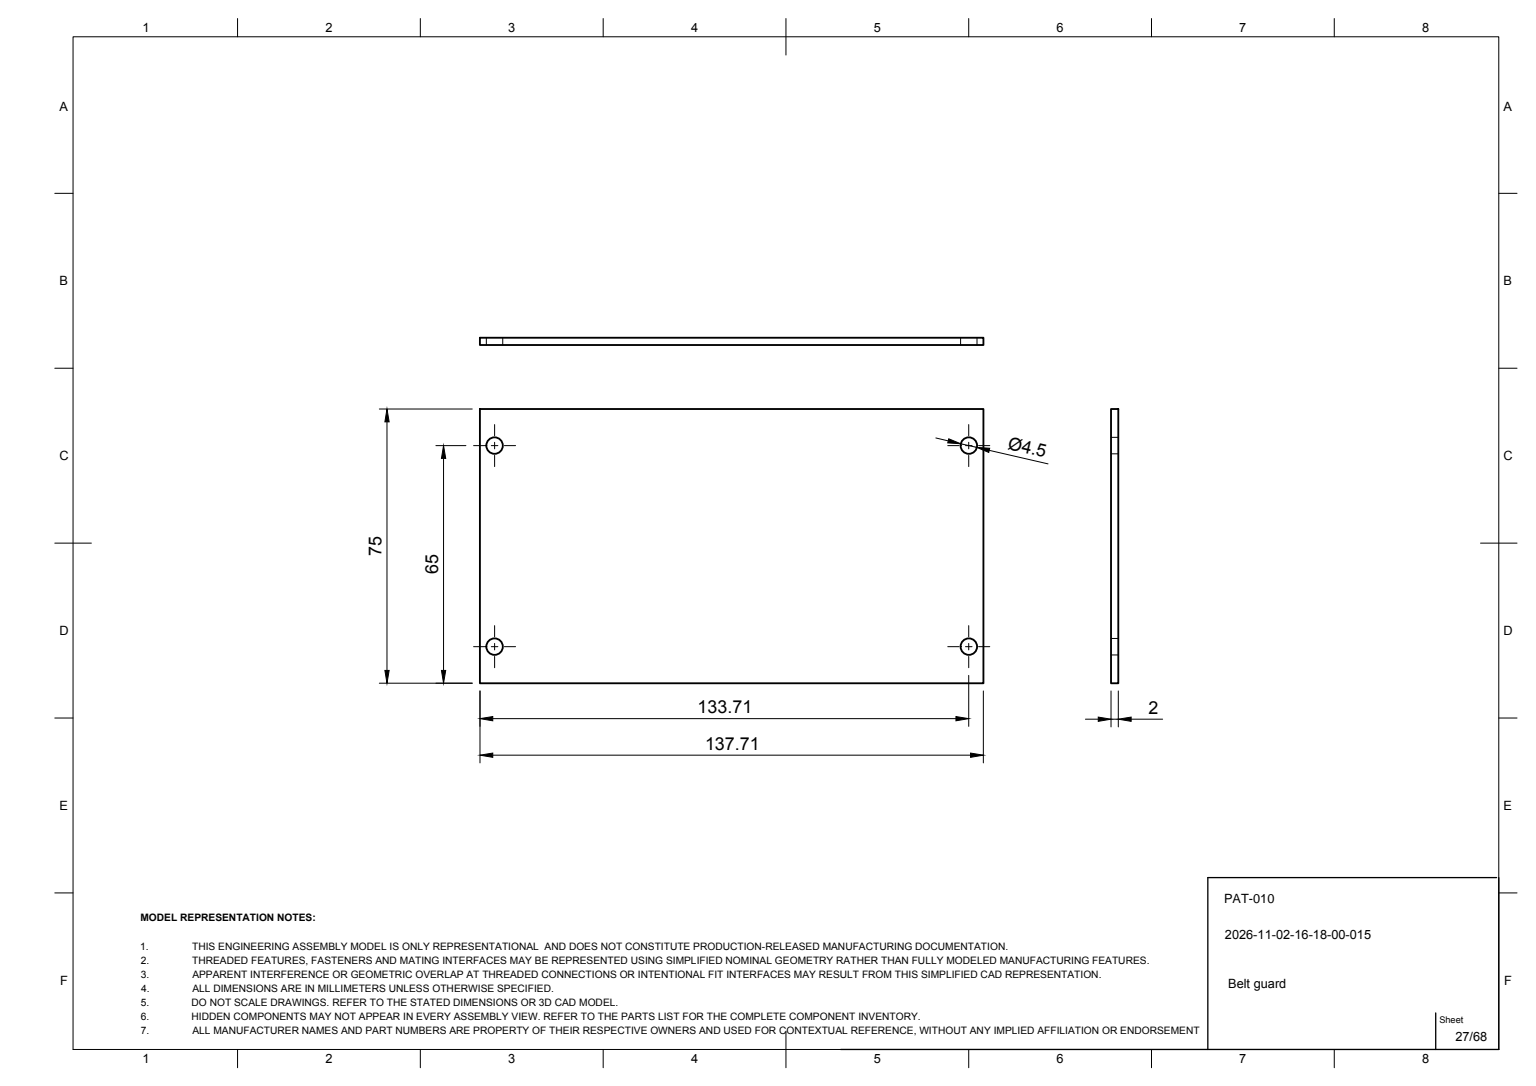
ISO-10303-21;
HEADER;
/* Generated by software containing ST-Developer
 * from STEP Tools, Inc. (www.steptools.com) 
 */

FILE_DESCRIPTION(
/* description */ ('Belt conveyor head drive unit'),
/* implementation_level */ '2;1');

FILE_NAME(
/* name */ 'Belt guard.step',
/* time_stamp */ '2026-10-28T03:26:19-07:00',
/* author */ (''),
/* organization */ (''),
/* preprocessor_version */ 'ST-DEVELOPER v20.2',
/* originating_system */ 'Autodesk Translation Framework v15.17.0.0',
/* authorisation */ '');

FILE_SCHEMA (('AUTOMOTIVE_DESIGN { 1 0 10303 214 3 1 1 }'));
ENDSEC;

DATA;
#10=MECHANICAL_DESIGN_GEOMETRIC_PRESENTATION_REPRESENTATION('',(#873),#27069);
#735=SHAPE_REPRESENTATION_RELATIONSHIP('SRR','None',#27379,#804);
#804=ADVANCED_BREP_SHAPE_REPRESENTATION('',(#958),#27021);
#873=STYLED_ITEM('',(#27804),#958);
#958=MANIFOLD_SOLID_BREP('Body1',#13738);
#1143=FACE_BOUND('',#2865,.T.);
#1144=FACE_BOUND('',#2866,.T.);
#1145=FACE_BOUND('',#2867,.T.);
#1146=FACE_BOUND('',#2868,.T.);
#1147=FACE_BOUND('',#2870,.T.);
#1148=FACE_BOUND('',#2871,.T.);
#1149=FACE_BOUND('',#2872,.T.);
#1150=FACE_BOUND('',#2873,.T.);
#1431=PLANE('',#15183);
#1432=PLANE('',#15184);
#1433=PLANE('',#15185);
#1434=PLANE('',#15186);
#1435=PLANE('',#15187);
#1436=PLANE('',#15188);
#1925=FACE_OUTER_BOUND('',#2856,.T.);
#1926=FACE_OUTER_BOUND('',#2857,.T.);
#1927=FACE_OUTER_BOUND('',#2858,.T.);
#1928=FACE_OUTER_BOUND('',#2859,.T.);
#1929=FACE_OUTER_BOUND('',#2860,.T.);
#1930=FACE_OUTER_BOUND('',#2861,.T.);
#1931=FACE_OUTER_BOUND('',#2862,.T.);
#1932=FACE_OUTER_BOUND('',#2863,.T.);
#1933=FACE_OUTER_BOUND('',#2864,.T.);
#1934=FACE_OUTER_BOUND('',#2869,.T.);
#2856=EDGE_LOOP('',(#10224,#10225,#10226,#10227));
#2857=EDGE_LOOP('',(#10228,#10229,#10230,#10231));
#2858=EDGE_LOOP('',(#10232,#10233,#10234,#10235));
#2859=EDGE_LOOP('',(#10236,#10237,#10238,#10239));
#2860=EDGE_LOOP('',(#10240,#10241,#10242,#10243));
#2861=EDGE_LOOP('',(#10244,#10245,#10246,#10247));
#2862=EDGE_LOOP('',(#10248,#10249,#10250,#10251));
#2863=EDGE_LOOP('',(#10252,#10253,#10254,#10255));
#2864=EDGE_LOOP('',(#10256,#10257,#10258,#10259));
#2865=EDGE_LOOP('',(#10260));
#2866=EDGE_LOOP('',(#10261));
#2867=EDGE_LOOP('',(#10262));
#2868=EDGE_LOOP('',(#10263));
#2869=EDGE_LOOP('',(#10264,#10265,#10266,#10267));
#2870=EDGE_LOOP('',(#10268));
#2871=EDGE_LOOP('',(#10269));
#2872=EDGE_LOOP('',(#10270));
#2873=EDGE_LOOP('',(#10271));
#3843=LINE('',#22350,#4635);
#3844=LINE('',#22356,#4636);
#3845=LINE('',#22362,#4637);
#3846=LINE('',#22368,#4638);
#3847=LINE('',#22373,#4639);
#3848=LINE('',#22375,#4640);
#3849=LINE('',#22377,#4641);
#3850=LINE('',#22378,#4642);
#3851=LINE('',#22381,#4643);
#3852=LINE('',#22383,#4644);
#3853=LINE('',#22384,#4645);
#3854=LINE('',#22387,#4646);
#3855=LINE('',#22389,#4647);
#3856=LINE('',#22390,#4648);
#3857=LINE('',#22392,#4649);
#3858=LINE('',#22393,#4650);
#4635=VECTOR('',#18001,0.225);
#4636=VECTOR('',#18008,0.225);
#4637=VECTOR('',#18015,0.225);
#4638=VECTOR('',#18022,0.225);
#4639=VECTOR('',#18027,1.);
#4640=VECTOR('',#18028,1.);
#4641=VECTOR('',#18029,1.);
#4642=VECTOR('',#18030,1.);
#4643=VECTOR('',#18033,1.);
#4644=VECTOR('',#18034,1.);
#4645=VECTOR('',#18035,1.);
#4646=VECTOR('',#18038,1.);
#4647=VECTOR('',#18039,1.);
#4648=VECTOR('',#18040,1.);
#4649=VECTOR('',#18043,1.);
#4650=VECTOR('',#18044,1.);
#5370=CIRCLE('',#15172,0.225);
#5371=CIRCLE('',#15173,0.225);
#5372=CIRCLE('',#15175,0.225);
#5373=CIRCLE('',#15176,0.225);
#5374=CIRCLE('',#15178,0.225);
#5375=CIRCLE('',#15179,0.225);
#5376=CIRCLE('',#15181,0.225);
#5377=CIRCLE('',#15182,0.225);
#6375=VERTEX_POINT('',#22347);
#6376=VERTEX_POINT('',#22349);
#6377=VERTEX_POINT('',#22353);
#6378=VERTEX_POINT('',#22355);
#6379=VERTEX_POINT('',#22359);
#6380=VERTEX_POINT('',#22361);
#6381=VERTEX_POINT('',#22365);
#6382=VERTEX_POINT('',#22367);
#6383=VERTEX_POINT('',#22371);
#6384=VERTEX_POINT('',#22372);
#6385=VERTEX_POINT('',#22374);
#6386=VERTEX_POINT('',#22376);
#6387=VERTEX_POINT('',#22380);
#6388=VERTEX_POINT('',#22382);
#6389=VERTEX_POINT('',#22386);
#6390=VERTEX_POINT('',#22388);
#7804=EDGE_CURVE('',#6375,#6375,#5370,.T.);
#7805=EDGE_CURVE('',#6375,#6376,#3843,.T.);
#7806=EDGE_CURVE('',#6376,#6376,#5371,.T.);
#7807=EDGE_CURVE('',#6377,#6377,#5372,.T.);
#7808=EDGE_CURVE('',#6377,#6378,#3844,.T.);
#7809=EDGE_CURVE('',#6378,#6378,#5373,.T.);
#7810=EDGE_CURVE('',#6379,#6379,#5374,.T.);
#7811=EDGE_CURVE('',#6379,#6380,#3845,.T.);
#7812=EDGE_CURVE('',#6380,#6380,#5375,.T.);
#7813=EDGE_CURVE('',#6381,#6381,#5376,.T.);
#7814=EDGE_CURVE('',#6381,#6382,#3846,.T.);
#7815=EDGE_CURVE('',#6382,#6382,#5377,.T.);
#7816=EDGE_CURVE('',#6383,#6384,#3847,.T.);
#7817=EDGE_CURVE('',#6383,#6385,#3848,.T.);
#7818=EDGE_CURVE('',#6386,#6385,#3849,.T.);
#7819=EDGE_CURVE('',#6384,#6386,#3850,.T.);
#7820=EDGE_CURVE('',#6384,#6387,#3851,.T.);
#7821=EDGE_CURVE('',#6388,#6386,#3852,.T.);
#7822=EDGE_CURVE('',#6387,#6388,#3853,.T.);
#7823=EDGE_CURVE('',#6387,#6389,#3854,.T.);
#7824=EDGE_CURVE('',#6390,#6388,#3855,.T.);
#7825=EDGE_CURVE('',#6389,#6390,#3856,.T.);
#7826=EDGE_CURVE('',#6389,#6383,#3857,.T.);
#7827=EDGE_CURVE('',#6385,#6390,#3858,.T.);
#10224=ORIENTED_EDGE('',*,*,#7804,.F.);
#10225=ORIENTED_EDGE('',*,*,#7805,.T.);
#10226=ORIENTED_EDGE('',*,*,#7806,.F.);
#10227=ORIENTED_EDGE('',*,*,#7805,.F.);
#10228=ORIENTED_EDGE('',*,*,#7807,.F.);
#10229=ORIENTED_EDGE('',*,*,#7808,.T.);
#10230=ORIENTED_EDGE('',*,*,#7809,.F.);
#10231=ORIENTED_EDGE('',*,*,#7808,.F.);
#10232=ORIENTED_EDGE('',*,*,#7810,.F.);
#10233=ORIENTED_EDGE('',*,*,#7811,.T.);
#10234=ORIENTED_EDGE('',*,*,#7812,.F.);
#10235=ORIENTED_EDGE('',*,*,#7811,.F.);
#10236=ORIENTED_EDGE('',*,*,#7813,.F.);
#10237=ORIENTED_EDGE('',*,*,#7814,.T.);
#10238=ORIENTED_EDGE('',*,*,#7815,.F.);
#10239=ORIENTED_EDGE('',*,*,#7814,.F.);
#10240=ORIENTED_EDGE('',*,*,#7816,.F.);
#10241=ORIENTED_EDGE('',*,*,#7817,.T.);
#10242=ORIENTED_EDGE('',*,*,#7818,.F.);
#10243=ORIENTED_EDGE('',*,*,#7819,.F.);
#10244=ORIENTED_EDGE('',*,*,#7820,.F.);
#10245=ORIENTED_EDGE('',*,*,#7819,.T.);
#10246=ORIENTED_EDGE('',*,*,#7821,.F.);
#10247=ORIENTED_EDGE('',*,*,#7822,.F.);
#10248=ORIENTED_EDGE('',*,*,#7823,.F.);
#10249=ORIENTED_EDGE('',*,*,#7822,.T.);
#10250=ORIENTED_EDGE('',*,*,#7824,.F.);
#10251=ORIENTED_EDGE('',*,*,#7825,.F.);
#10252=ORIENTED_EDGE('',*,*,#7826,.F.);
#10253=ORIENTED_EDGE('',*,*,#7825,.T.);
#10254=ORIENTED_EDGE('',*,*,#7827,.F.);
#10255=ORIENTED_EDGE('',*,*,#7817,.F.);
#10256=ORIENTED_EDGE('',*,*,#7827,.T.);
#10257=ORIENTED_EDGE('',*,*,#7824,.T.);
#10258=ORIENTED_EDGE('',*,*,#7821,.T.);
#10259=ORIENTED_EDGE('',*,*,#7818,.T.);
#10260=ORIENTED_EDGE('',*,*,#7806,.T.);
#10261=ORIENTED_EDGE('',*,*,#7809,.T.);
#10262=ORIENTED_EDGE('',*,*,#7812,.T.);
#10263=ORIENTED_EDGE('',*,*,#7815,.T.);
#10264=ORIENTED_EDGE('',*,*,#7826,.T.);
#10265=ORIENTED_EDGE('',*,*,#7816,.T.);
#10266=ORIENTED_EDGE('',*,*,#7820,.T.);
#10267=ORIENTED_EDGE('',*,*,#7823,.T.);
#10268=ORIENTED_EDGE('',*,*,#7804,.T.);
#10269=ORIENTED_EDGE('',*,*,#7807,.T.);
#10270=ORIENTED_EDGE('',*,*,#7810,.T.);
#10271=ORIENTED_EDGE('',*,*,#7813,.T.);
#12670=CYLINDRICAL_SURFACE('',#15171,0.225);
#12671=CYLINDRICAL_SURFACE('',#15174,0.225);
#12672=CYLINDRICAL_SURFACE('',#15177,0.225);
#12673=CYLINDRICAL_SURFACE('',#15180,0.225);
#13204=ADVANCED_FACE('',(#1925),#12670,.F.);
#13205=ADVANCED_FACE('',(#1926),#12671,.F.);
#13206=ADVANCED_FACE('',(#1927),#12672,.F.);
#13207=ADVANCED_FACE('',(#1928),#12673,.F.);
#13208=ADVANCED_FACE('',(#1929),#1431,.T.);
#13209=ADVANCED_FACE('',(#1930),#1432,.T.);
#13210=ADVANCED_FACE('',(#1931),#1433,.T.);
#13211=ADVANCED_FACE('',(#1932),#1434,.T.);
#13212=ADVANCED_FACE('',(#1933,#1143,#1144,#1145,#1146),#1435,.T.);
#13213=ADVANCED_FACE('',(#1934,#1147,#1148,#1149,#1150),#1436,.F.);
#13738=CLOSED_SHELL('',(#13204,#13205,#13206,#13207,#13208,#13209,#13210,
#13211,#13212,#13213));
#15170=AXIS2_PLACEMENT_3D('',#22345,#17995,#17996);
#15171=AXIS2_PLACEMENT_3D('',#22346,#17997,#17998);
#15172=AXIS2_PLACEMENT_3D('',#22348,#17999,#18000);
#15173=AXIS2_PLACEMENT_3D('',#22351,#18002,#18003);
#15174=AXIS2_PLACEMENT_3D('',#22352,#18004,#18005);
#15175=AXIS2_PLACEMENT_3D('',#22354,#18006,#18007);
#15176=AXIS2_PLACEMENT_3D('',#22357,#18009,#18010);
#15177=AXIS2_PLACEMENT_3D('',#22358,#18011,#18012);
#15178=AXIS2_PLACEMENT_3D('',#22360,#18013,#18014);
#15179=AXIS2_PLACEMENT_3D('',#22363,#18016,#18017);
#15180=AXIS2_PLACEMENT_3D('',#22364,#18018,#18019);
#15181=AXIS2_PLACEMENT_3D('',#22366,#18020,#18021);
#15182=AXIS2_PLACEMENT_3D('',#22369,#18023,#18024);
#15183=AXIS2_PLACEMENT_3D('',#22370,#18025,#18026);
#15184=AXIS2_PLACEMENT_3D('',#22379,#18031,#18032);
#15185=AXIS2_PLACEMENT_3D('',#22385,#18036,#18037);
#15186=AXIS2_PLACEMENT_3D('',#22391,#18041,#18042);
#15187=AXIS2_PLACEMENT_3D('',#22394,#18045,#18046);
#15188=AXIS2_PLACEMENT_3D('',#22395,#18047,#18048);
#17995=DIRECTION('axis',(0.,0.,1.));
#17996=DIRECTION('refdir',(1.,0.,0.));
#17997=DIRECTION('center_axis',(0.,1.,0.));
#17998=DIRECTION('ref_axis',(1.,0.,0.));
#17999=DIRECTION('center_axis',(0.,1.,0.));
#18000=DIRECTION('ref_axis',(1.,0.,0.));
#18001=DIRECTION('',(0.,1.,0.));
#18002=DIRECTION('center_axis',(0.,-1.,0.));
#18003=DIRECTION('ref_axis',(1.,0.,0.));
#18004=DIRECTION('center_axis',(0.,1.,0.));
#18005=DIRECTION('ref_axis',(1.,0.,0.));
#18006=DIRECTION('center_axis',(0.,1.,0.));
#18007=DIRECTION('ref_axis',(1.,0.,0.));
#18008=DIRECTION('',(0.,1.,0.));
#18009=DIRECTION('center_axis',(0.,-1.,0.));
#18010=DIRECTION('ref_axis',(1.,0.,0.));
#18011=DIRECTION('center_axis',(0.,1.,0.));
#18012=DIRECTION('ref_axis',(1.,0.,0.));
#18013=DIRECTION('center_axis',(0.,1.,0.));
#18014=DIRECTION('ref_axis',(1.,0.,0.));
#18015=DIRECTION('',(0.,1.,0.));
#18016=DIRECTION('center_axis',(0.,-1.,0.));
#18017=DIRECTION('ref_axis',(1.,0.,0.));
#18018=DIRECTION('center_axis',(0.,1.,0.));
#18019=DIRECTION('ref_axis',(1.,0.,0.));
#18020=DIRECTION('center_axis',(0.,1.,0.));
#18021=DIRECTION('ref_axis',(1.,0.,0.));
#18022=DIRECTION('',(0.,1.,0.));
#18023=DIRECTION('center_axis',(0.,-1.,0.));
#18024=DIRECTION('ref_axis',(1.,0.,0.));
#18025=DIRECTION('center_axis',(-1.,0.,0.));
#18026=DIRECTION('ref_axis',(0.,0.,1.));
#18027=DIRECTION('',(0.,0.,-1.));
#18028=DIRECTION('',(0.,1.,0.));
#18029=DIRECTION('',(0.,0.,1.));
#18030=DIRECTION('',(0.,1.,0.));
#18031=DIRECTION('center_axis',(0.,0.,-1.));
#18032=DIRECTION('ref_axis',(-1.,0.,0.));
#18033=DIRECTION('',(1.,0.,0.));
#18034=DIRECTION('',(-1.,0.,0.));
#18035=DIRECTION('',(0.,1.,0.));
#18036=DIRECTION('center_axis',(1.,0.,0.));
#18037=DIRECTION('ref_axis',(0.,0.,-1.));
#18038=DIRECTION('',(0.,0.,1.));
#18039=DIRECTION('',(0.,0.,-1.));
#18040=DIRECTION('',(0.,1.,0.));
#18041=DIRECTION('center_axis',(0.,0.,1.));
#18042=DIRECTION('ref_axis',(1.,0.,0.));
#18043=DIRECTION('',(-1.,0.,0.));
#18044=DIRECTION('',(1.,0.,0.));
#18045=DIRECTION('center_axis',(0.,1.,0.));
#18046=DIRECTION('ref_axis',(0.,0.,1.));
#18047=DIRECTION('center_axis',(0.,1.,0.));
#18048=DIRECTION('ref_axis',(1.,0.,0.));
#22345=CARTESIAN_POINT('',(0.,0.,0.));
#22346=CARTESIAN_POINT('Origin',(9.97091003018116,-6.3,4.5));
#22347=CARTESIAN_POINT('',(9.74591003018116,-6.2,4.5));
#22348=CARTESIAN_POINT('Origin',(9.97091003018116,-6.2,4.5));
#22349=CARTESIAN_POINT('',(9.74591003018116,-6.,4.5));
#22350=CARTESIAN_POINT('',(9.74591003018116,-6.3,4.5));
#22351=CARTESIAN_POINT('Origin',(9.97091003018116,-6.,4.5));
#22352=CARTESIAN_POINT('Origin',(-3.,-6.3,10.));
#22353=CARTESIAN_POINT('',(-3.225,-6.2,10.));
#22354=CARTESIAN_POINT('Origin',(-3.,-6.2,10.));
#22355=CARTESIAN_POINT('',(-3.225,-6.,10.));
#22356=CARTESIAN_POINT('',(-3.225,-6.3,10.));
#22357=CARTESIAN_POINT('Origin',(-3.,-6.,10.));
#22358=CARTESIAN_POINT('Origin',(-3.,-6.3,4.5));
#22359=CARTESIAN_POINT('',(-3.225,-6.2,4.5));
#22360=CARTESIAN_POINT('Origin',(-3.,-6.2,4.5));
#22361=CARTESIAN_POINT('',(-3.225,-6.,4.5));
#22362=CARTESIAN_POINT('',(-3.225,-6.3,4.5));
#22363=CARTESIAN_POINT('Origin',(-3.,-6.,4.5));
#22364=CARTESIAN_POINT('Origin',(9.97091003018116,-6.3,10.));
#22365=CARTESIAN_POINT('',(9.74591003018116,-6.2,10.));
#22366=CARTESIAN_POINT('Origin',(9.97091003018116,-6.2,10.));
#22367=CARTESIAN_POINT('',(9.74591003018116,-6.,10.));
#22368=CARTESIAN_POINT('',(9.74591003018116,-6.3,10.));
#22369=CARTESIAN_POINT('Origin',(9.97091003018116,-6.,10.));
#22370=CARTESIAN_POINT('Origin',(-3.4,-6.2,3.5));
#22371=CARTESIAN_POINT('',(-3.4,-6.2,11.));
#22372=CARTESIAN_POINT('',(-3.4,-6.2,3.5));
#22373=CARTESIAN_POINT('',(-3.4,-6.2,11.));
#22374=CARTESIAN_POINT('',(-3.4,-6.,11.));
#22375=CARTESIAN_POINT('',(-3.4,-6.2,11.));
#22376=CARTESIAN_POINT('',(-3.4,-6.,3.5));
#22377=CARTESIAN_POINT('',(-3.4,-6.,11.));
#22378=CARTESIAN_POINT('',(-3.4,-6.2,3.5));
#22379=CARTESIAN_POINT('Origin',(10.3709100301812,-6.2,3.5));
#22380=CARTESIAN_POINT('',(10.3709100301812,-6.2,3.5));
#22381=CARTESIAN_POINT('',(-3.4,-6.2,3.5));
#22382=CARTESIAN_POINT('',(10.3709100301812,-6.,3.5));
#22383=CARTESIAN_POINT('',(-3.4,-6.,3.5));
#22384=CARTESIAN_POINT('',(10.3709100301812,-6.2,3.5));
#22385=CARTESIAN_POINT('Origin',(10.3709100301812,-6.2,11.));
#22386=CARTESIAN_POINT('',(10.3709100301812,-6.2,11.));
#22387=CARTESIAN_POINT('',(10.3709100301812,-6.2,3.5));
#22388=CARTESIAN_POINT('',(10.3709100301812,-6.,11.));
#22389=CARTESIAN_POINT('',(10.3709100301812,-6.,3.5));
#22390=CARTESIAN_POINT('',(10.3709100301812,-6.2,11.));
#22391=CARTESIAN_POINT('Origin',(-3.4,-6.2,11.));
#22392=CARTESIAN_POINT('',(10.3709100301812,-6.2,11.));
#22393=CARTESIAN_POINT('',(10.3709100301812,-6.,11.));
#22394=CARTESIAN_POINT('Origin',(3.48545501509058,-6.,7.25));
#22395=CARTESIAN_POINT('Origin',(3.48545501509058,-6.2,7.25));
#26944=UNCERTAINTY_MEASURE_WITH_UNIT(LENGTH_MEASURE(0.001),#27070,
'DISTANCE_ACCURACY_VALUE',
'Maximum model space distance between geometric entities at asserted c
onnectivities');
#26992=UNCERTAINTY_MEASURE_WITH_UNIT(LENGTH_MEASURE(0.001),#27070,
'DISTANCE_ACCURACY_VALUE',
'Maximum model space distance between geometric entities at asserted c
onnectivities');
#27021=(
GEOMETRIC_REPRESENTATION_CONTEXT(3)
GLOBAL_UNCERTAINTY_ASSIGNED_CONTEXT((#26944))
GLOBAL_UNIT_ASSIGNED_CONTEXT((#27070,#27072,#27073))
REPRESENTATION_CONTEXT('','3D')
);
#27069=(
GEOMETRIC_REPRESENTATION_CONTEXT(3)
GLOBAL_UNCERTAINTY_ASSIGNED_CONTEXT((#26992))
GLOBAL_UNIT_ASSIGNED_CONTEXT((#27070,#27072,#27073))
REPRESENTATION_CONTEXT('','3D')
);
#27070=(
LENGTH_UNIT()
NAMED_UNIT(*)
SI_UNIT(.CENTI.,.METRE.)
);
#27072=(
NAMED_UNIT(*)
PLANE_ANGLE_UNIT()
SI_UNIT($,.RADIAN.)
);
#27073=(
NAMED_UNIT(*)
SI_UNIT($,.STERADIAN.)
SOLID_ANGLE_UNIT()
);
#27102=SHAPE_DEFINITION_REPRESENTATION(#27178,#27379);
#27178=PRODUCT_DEFINITION_SHAPE('',$,#27456);
#27379=SHAPE_REPRESENTATION('',(#15170),#27021);
#27427=PRODUCT_DEFINITION_CONTEXT('part definition',#27657,'design');
#27456=PRODUCT_DEFINITION('Belt guard','Belt guard',#27532,#27427);
#27532=PRODUCT_DEFINITION_FORMATION('',$,#27687);
#27657=APPLICATION_CONTEXT(
'Core Data for Automotive Mechanical Design Process');
#27658=PRODUCT_CONTEXT('part definition',#27657,'mechanical');
#27687=PRODUCT('Belt guard','Belt guard','Belt guard',(#27658));
#27798=COLOUR_RGB('Black',0.12,0.14,0.17);
#27799=FILL_AREA_STYLE_COLOUR('',#27798);
#27800=FILL_AREA_STYLE('',(#27799));
#27801=SURFACE_STYLE_FILL_AREA(#27800);
#27802=SURFACE_SIDE_STYLE('',(#27801));
#27803=SURFACE_STYLE_USAGE(.BOTH.,#27802);
#27804=PRESENTATION_STYLE_ASSIGNMENT((#27803));
ENDSEC;
END-ISO-10303-21;
